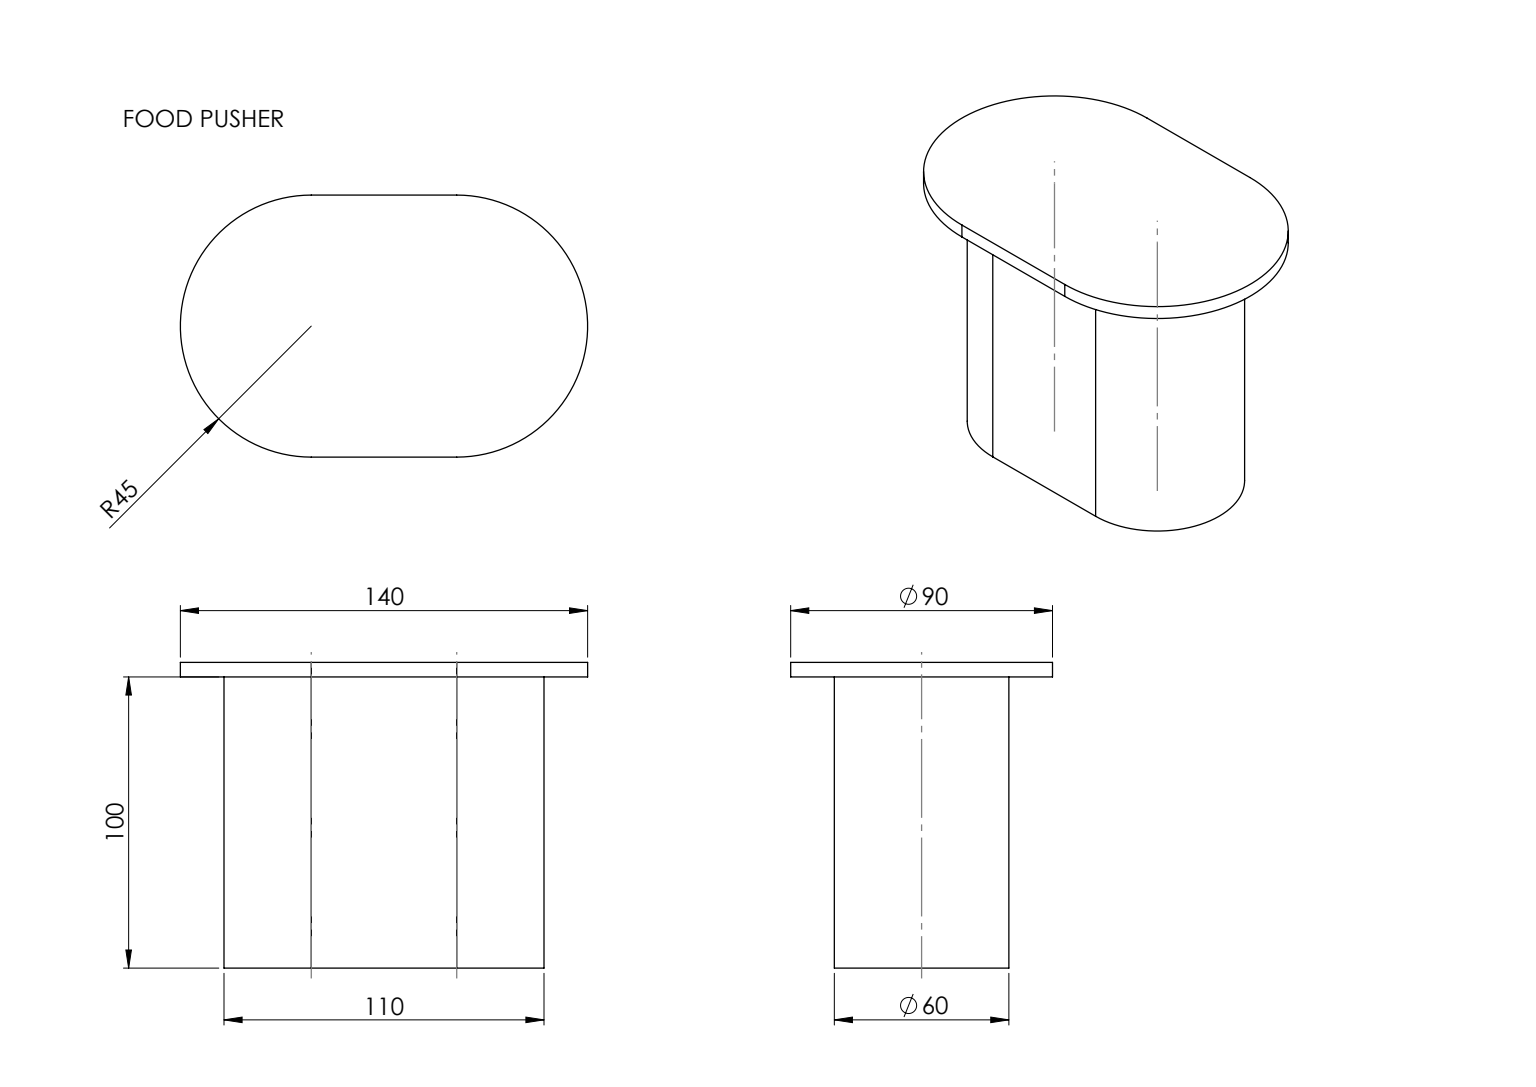
ISO-10303-21;
HEADER;
FILE_DESCRIPTION (('STEP AP214'),
    '1' );
FILE_NAME ('Food Pusher.step',
    '2026-10-08T14:59:03',
    ( '' ),
    ( '' ),
    'SwSTEP 2.0',
    'SolidWorks 2026',
    '' );
FILE_SCHEMA (( 'AUTOMOTIVE_DESIGN' ));
ENDSEC;

DATA;
#34=DIRECTION ( 'NONE',  ( 0.000000000000000000, -0.000000000000000000, 1.000000000000000000 ) ) ;
#70=CARTESIAN_POINT ( 'NONE',  ( -25.00000000000000000, 347.0000000000000568, -88.00000000000000000 ) ) ;
#77=PRESENTATION_STYLE_ASSIGNMENT (( #1089 ) ) ;
#97=CARTESIAN_POINT ( 'NONE',  ( 25.00000000000000000, 445.0000000000000568, -59.99999999999999289 ) ) ;
#102=PRODUCT ( 'Food Pusher', 'Food Pusher', '', ( #178 ) ) ;
#125=AXIS2_PLACEMENT_3D ( 'NONE', #9417, #9481, #11434 ) ;
#140=EDGE_CURVE ( 'NONE', #6671, #381, #10679, .T. ) ;
#178=PRODUCT_CONTEXT ( 'NONE', #12278, 'mechanical' ) ;
#190=DIRECTION ( 'NONE',  ( 0.000000000000000000, 1.000000000000000000, 0.000000000000000000 ) ) ;
#266=ORIENTED_EDGE ( 'NONE', *, *, #6038, .T. ) ;
#269=PRODUCT_DEFINITION_CONTEXT ( 'detailed design', #4862, 'design' ) ;
#304=EDGE_CURVE ( 'NONE', #3140, #9041, #7672, .T. ) ;
#351=EDGE_CURVE ( 'NONE', #5322, #7972, #10426, .T. ) ;
#367=LINE ( 'NONE', #11973, #3584 ) ;
#381=VERTEX_POINT ( 'NONE', #5888 ) ;
#385=AXIS2_PLACEMENT_3D ( 'NONE', #9164, #2752, #5571 ) ;
#431=ORIENTED_EDGE ( 'NONE', *, *, #7084, .F. ) ;
#458=CARTESIAN_POINT ( 'NONE',  ( -25.00000000000000000, 345.0000000000000568, -29.99999999999999289 ) ) ;
#475=CARTESIAN_POINT ( 'NONE',  ( 25.00000000000000355, 347.0000000000000568, -31.99999999999998579 ) ) ;
#481=ADVANCED_FACE ( 'NONE', ( #10318 ), #11460, .T. ) ;
#530=UNCERTAINTY_MEASURE_WITH_UNIT (LENGTH_MEASURE( 1.000000000000000082E-05 ), #1165, 'distance_accuracy_value', 'NONE');
#538=EDGE_CURVE ( 'NONE', #3006, #5730, #8937, .T. ) ;
#543=BREP_WITH_VOIDS ( 'NONE', #9857, ( #2440 ) );
#547=ORIENTED_EDGE ( 'NONE', *, *, #6712, .T. ) ;
#549=LINE ( 'NONE', #7222, #4086 ) ;
#581=ORIENTED_EDGE ( 'NONE', *, *, #4046, .F. ) ;
#591=ORIENTED_EDGE ( 'NONE', *, *, #140, .T. ) ;
#598=DIRECTION ( 'NONE',  ( 1.000000000000000000, 0.000000000000000000, 6.938893903907229610E-17 ) ) ;
#684=CARTESIAN_POINT ( 'NONE',  ( 25.00000000000000000, 445.0000000000000568, -59.99999999999999289 ) ) ;
#689=LINE ( 'NONE', #7424, #4842 ) ;
#727=AXIS2_PLACEMENT_3D ( 'NONE', #9151, #8407, #2620 ) ;
#755=FACE_OUTER_BOUND ( 'NONE', #1895, .T. ) ;
#758=CARTESIAN_POINT ( 'NONE',  ( -25.00000000000000000, 345.0000000000000568, -90.00000000000000000 ) ) ;
#776=MECHANICAL_DESIGN_GEOMETRIC_PRESENTATION_REPRESENTATION('',(#5155),#10705);
#836=ORIENTED_EDGE ( 'NONE', *, *, #7826, .F. ) ;
#837=DIRECTION ( 'NONE',  ( 0.000000000000000000, -0.000000000000000000, 1.000000000000000000 ) ) ;
#869=PRODUCT_DEFINITION ( 'UNKNOWN', '', #3750, #269 ) ;
#915=LINE ( 'NONE', #11450, #4998 ) ;
#940=LINE ( 'NONE', #12287, #7026 ) ;
#961=ORIENTED_EDGE ( 'NONE', *, *, #5528, .F. ) ;
#999=CARTESIAN_POINT ( 'NONE',  ( -25.00000000000000000, 445.0000000000000568, -29.99999999999999289 ) ) ;
#1065=CYLINDRICAL_SURFACE ( 'NONE', #6806, 44.99999999999999289 ) ;
#1077=FACE_OUTER_BOUND ( 'NONE', #5495, .T. ) ;
#1089=SURFACE_STYLE_USAGE ( .BOTH. , #2893 ) ;
#1095=VERTEX_POINT ( 'NONE', #1645 ) ;
#1102=AXIS2_PLACEMENT_3D ( 'NONE', #5202, #8863, #11996 ) ;
#1119=VECTOR ( 'NONE', #10886, 1000.000000000000000 ) ;
#1120=ORIENTED_EDGE ( 'NONE', *, *, #11826, .T. ) ;
#1165=( LENGTH_UNIT ( ) NAMED_UNIT ( * ) SI_UNIT ( .MILLI., .METRE. ) );
#1181=ADVANCED_FACE ( 'NONE', ( #10357 ), #10419, .F. ) ;
#1201=CARTESIAN_POINT ( 'NONE',  ( 25.00000000000000000, 570.2996408614167194, -59.99999999999999289 ) ) ;
#1219=DIRECTION ( 'NONE',  ( 0.000000000000000000, 0.000000000000000000, 1.000000000000000000 ) ) ;
#1241=ORIENTED_EDGE ( 'NONE', *, *, #2131, .F. ) ;
#1287=CARTESIAN_POINT ( 'NONE',  ( -25.00000000000000000, 570.2996408614167194, -29.99999999999999289 ) ) ;
#1303=ORIENTED_EDGE ( 'NONE', *, *, #5273, .F. ) ;
#1345=EDGE_CURVE ( 'NONE', #11537, #3527, #3608, .T. ) ;
#1374=VERTEX_POINT ( 'NONE', #8728 ) ;
#1396=EDGE_CURVE ( 'NONE', #11537, #1374, #6932, .T. ) ;
#1458=ORIENTED_EDGE ( 'NONE', *, *, #7606, .F. ) ;
#1492=DIRECTION ( 'NONE',  ( 1.000000000000000000, 0.000000000000000000, -0.000000000000000000 ) ) ;
#1503=EDGE_LOOP ( 'NONE', ( #8693, #4343, #10905, #836 ) ) ;
#1508=ORIENTED_EDGE ( 'NONE', *, *, #4461, .F. ) ;
#1585=( GEOMETRIC_REPRESENTATION_CONTEXT ( 3 ) GLOBAL_UNCERTAINTY_ASSIGNED_CONTEXT ( ( #530 ) ) GLOBAL_UNIT_ASSIGNED_CONTEXT ( ( #1165, #7827, #5035 ) ) REPRESENTATION_CONTEXT ( 'NONE', 'WORKASPACE' ) );
#1599=VECTOR ( 'NONE', #1889, 1000.000000000000000 ) ;
#1601=DIRECTION ( 'NONE',  ( 1.000000000000000000, -0.000000000000000000, 6.938893903907228378E-17 ) ) ;
#1612=AXIS2_PLACEMENT_3D ( 'NONE', #9562, #7823, #5032 ) ;
#1636=EDGE_LOOP ( 'NONE', ( #5230, #2543, #266, #6949 ) ) ;
#1645=CARTESIAN_POINT ( 'NONE',  ( 25.00000000000000355, 445.0000000000000568, -31.99999999999998579 ) ) ;
#1650=CARTESIAN_POINT ( 'NONE',  ( -25.00000000000000000, 450.0000000000000568, -14.99999999999999289 ) ) ;
#1651=VECTOR ( 'NONE', #598, 1000.000000000000000 ) ;
#1670=CARTESIAN_POINT ( 'NONE',  ( -25.00000000000000000, 445.0000000000000568, -59.99999999999999289 ) ) ;
#1734=VERTEX_POINT ( 'NONE', #758 ) ;
#1741=ADVANCED_FACE ( 'NONE', ( #7427 ), #8571, .F. ) ;
#1743=DIRECTION ( 'NONE',  ( 0.000000000000000000, 0.000000000000000000, 1.000000000000000000 ) ) ;
#1772=ORIENTED_EDGE ( 'NONE', *, *, #6771, .T. ) ;
#1777=ORIENTED_EDGE ( 'NONE', *, *, #8505, .T. ) ;
#1807=EDGE_LOOP ( 'NONE', ( #2058, #5789, #5095, #6562 ) ) ;
#1809=PLANE ( 'NONE',  #727 ) ;
#1819=VECTOR ( 'NONE', #2010, 1000.000000000000000 ) ;
#1848=DIRECTION ( 'NONE',  ( -0.000000000000000000, -1.000000000000000000, -0.000000000000000000 ) ) ;
#1875=CIRCLE ( 'NONE', #11248, 30.00000000000000355 ) ;
#1889=DIRECTION ( 'NONE',  ( -1.000000000000000000, 0.000000000000000000, 0.000000000000000000 ) ) ;
#1895=EDGE_LOOP ( 'NONE', ( #3084, #6423, #581, #4488 ) ) ;
#1908=ORIENTED_EDGE ( 'NONE', *, *, #1345, .T. ) ;
#1955=DIRECTION ( 'NONE',  ( -0.000000000000000000, -1.000000000000000000, -0.000000000000000000 ) ) ;
#2010=DIRECTION ( 'NONE',  ( -0.000000000000000000, -1.000000000000000000, -0.000000000000000000 ) ) ;
#2020=AXIS2_PLACEMENT_3D ( 'NONE', #97, #11523, #34 ) ;
#2058=ORIENTED_EDGE ( 'NONE', *, *, #5528, .T. ) ;
#2070=EDGE_LOOP ( 'NONE', ( #3023, #6435, #6345, #7354 ) ) ;
#2113=VERTEX_POINT ( 'NONE', #3709 ) ;
#2131=EDGE_CURVE ( 'NONE', #10138, #2113, #915, .T. ) ;
#2158=EDGE_CURVE ( 'NONE', #1095, #5322, #3373, .T. ) ;
#2170=EDGE_LOOP ( 'NONE', ( #1120, #3244, #10555, #5195 ) ) ;
#2190=CARTESIAN_POINT ( 'NONE',  ( 25.00000000000000000, 450.0000000000000568, -14.99999999999998934 ) ) ;
#2237=CARTESIAN_POINT ( 'NONE',  ( -24.99999999999999645, 450.0000000000000568, -105.0000000000000000 ) ) ;
#2338=FILL_AREA_STYLE_COLOUR ( '', #6280 ) ;
#2364=ADVANCED_FACE ( 'NONE', ( #9805 ), #3210, .T. ) ;
#2396=AXIS2_PLACEMENT_3D ( 'NONE', #8499, #10502, #12320 ) ;
#2440=ORIENTED_CLOSED_SHELL ( 'NONE', *, #12071, .F. );
#2466=ADVANCED_FACE ( 'NONE', ( #6560 ), #4626, .T. ) ;
#2543=ORIENTED_EDGE ( 'NONE', *, *, #9022, .T. ) ;
#2565=EDGE_LOOP ( 'NONE', ( #6905, #5701, #7059, #11308 ) ) ;
#2620=DIRECTION ( 'NONE',  ( 0.000000000000000000, -0.000000000000000000, 1.000000000000000000 ) ) ;
#2647=CARTESIAN_POINT ( 'NONE',  ( -25.00000000000000000, 347.0000000000000568, -59.99999999999999289 ) ) ;
#2657=ADVANCED_FACE ( 'NONE', ( #5934 ), #8665, .F. ) ;
#2699=ORIENTED_EDGE ( 'NONE', *, *, #2131, .T. ) ;
#2752=DIRECTION ( 'NONE',  ( 6.938893903907228378E-17, 0.000000000000000000, -1.000000000000000000 ) ) ;
#2767=DIRECTION ( 'NONE',  ( 0.000000000000000000, 0.000000000000000000, 1.000000000000000000 ) ) ;
#2783=DIRECTION ( 'NONE',  ( 0.000000000000000000, 0.000000000000000000, 1.000000000000000000 ) ) ;
#2795=VECTOR ( 'NONE', #3014, 1000.000000000000000 ) ;
#2811=ORIENTED_EDGE ( 'NONE', *, *, #4159, .F. ) ;
#2814=AXIS2_PLACEMENT_3D ( 'NONE', #4066, #190, #5937 ) ;
#2824=ORIENTED_EDGE ( 'NONE', *, *, #304, .F. ) ;
#2831=EDGE_LOOP ( 'NONE', ( #7123, #8086, #11427, #1508 ) ) ;
#2832=FILL_AREA_STYLE ('',( #5769 ) ) ;
#2835=AXIS2_PLACEMENT_3D ( 'NONE', #6137, #6950, #1219 ) ;
#2837=CARTESIAN_POINT ( 'NONE',  ( 25.00000000000000000, 445.0000000000000568, -59.99999999999999289 ) ) ;
#2893=SURFACE_SIDE_STYLE ('',( #6634 ) ) ;
#2902=DIRECTION ( 'NONE',  ( -0.000000000000000000, -1.000000000000000000, -0.000000000000000000 ) ) ;
#2931=LINE ( 'NONE', #3988, #5877 ) ;
#2943=CARTESIAN_POINT ( 'NONE',  ( -24.99999999999999289, 450.0000000000000568, -14.99999999999999289 ) ) ;
#2957=SHAPE_REPRESENTATION_RELATIONSHIP ( 'NONE' , 'NONE' ,  #8876, #6166 ) ;
#3006=VERTEX_POINT ( 'NONE', #999 ) ;
#3014=DIRECTION ( 'NONE',  ( -1.000000000000000000, 0.000000000000000000, 0.000000000000000000 ) ) ;
#3023=ORIENTED_EDGE ( 'NONE', *, *, #7075, .T. ) ;
#3084=ORIENTED_EDGE ( 'NONE', *, *, #2158, .T. ) ;
#3105=ORIENTED_EDGE ( 'NONE', *, *, #11826, .F. ) ;
#3127=ORIENTED_EDGE ( 'NONE', *, *, #1396, .F. ) ;
#3140=VERTEX_POINT ( 'NONE', #4795 ) ;
#3155=DIRECTION ( 'NONE',  ( -0.000000000000000000, -1.000000000000000000, -0.000000000000000000 ) ) ;
#3210=PLANE ( 'NONE',  #10957 ) ;
#3225=DIRECTION ( 'NONE',  ( 0.000000000000000000, -0.000000000000000000, 1.000000000000000000 ) ) ;
#3244=ORIENTED_EDGE ( 'NONE', *, *, #8505, .F. ) ;
#3249=DIRECTION ( 'NONE',  ( 0.000000000000000000, 0.000000000000000000, -1.000000000000000000 ) ) ;
#3251=CIRCLE ( 'NONE', #4048, 45.00000000000000000 ) ;
#3291=VECTOR ( 'NONE', #5624, 1000.000000000000000 ) ;
#3305=AXIS2_PLACEMENT_3D ( 'NONE', #9278, #11039, #5620 ) ;
#3318=DIRECTION ( 'NONE',  ( -0.000000000000000000, -1.000000000000000000, -0.000000000000000000 ) ) ;
#3326=DIRECTION ( 'NONE',  ( -0.000000000000000000, -1.000000000000000000, -0.000000000000000000 ) ) ;
#3357=EDGE_CURVE ( 'NONE', #5022, #9737, #12322, .T. ) ;
#3373=CIRCLE ( 'NONE', #2396, 28.00000000000000355 ) ;
#3436=VERTEX_POINT ( 'NONE', #5463 ) ;
#3456=CIRCLE ( 'NONE', #9811, 45.00000000000000000 ) ;
#3480=DIRECTION ( 'NONE',  ( 0.000000000000000000, 0.000000000000000000, 1.000000000000000000 ) ) ;
#3527=VERTEX_POINT ( 'NONE', #3959 ) ;
#3535=CARTESIAN_POINT ( 'NONE',  ( -25.00000000000000000, 347.0000000000000568, -31.99999999999999289 ) ) ;
#3554=CYLINDRICAL_SURFACE ( 'NONE', #5641, 28.00000000000000355 ) ;
#3558=CARTESIAN_POINT ( 'NONE',  ( 25.00000000000000000, 347.0000000000000568, -59.99999999999999289 ) ) ;
#3584=VECTOR ( 'NONE', #4173, 1000.000000000000000 ) ;
#3608=CIRCLE ( 'NONE', #2814, 45.00000000000000000 ) ;
#3620=FACE_OUTER_BOUND ( 'NONE', #7230, .T. ) ;
#3645=( LENGTH_UNIT ( ) NAMED_UNIT ( * ) SI_UNIT ( .MILLI., .METRE. ) );
#3649=CARTESIAN_POINT ( 'NONE',  ( -25.00000000000000000, 445.0000000000000568, -31.99999999999999289 ) ) ;
#3695=LINE ( 'NONE', #6513, #8088 ) ;
#3701=( NAMED_UNIT ( * ) SI_UNIT ( $, .STERADIAN. ) SOLID_ANGLE_UNIT ( ) );
#3709=CARTESIAN_POINT ( 'NONE',  ( -25.00000000000000000, 445.0000000000000568, -14.99999999999999289 ) ) ;
#3711=LINE ( 'NONE', #6336, #11290 ) ;
#3718=ADVANCED_FACE ( 'NONE', ( #1077 ), #4753, .T. ) ;
#3729=CARTESIAN_POINT ( 'NONE',  ( -25.00000000000000000, 445.0000000000000568, -29.99999999999999289 ) ) ;
#3735=VERTEX_POINT ( 'NONE', #4885 ) ;
#3750=PRODUCT_DEFINITION_FORMATION_WITH_SPECIFIED_SOURCE ( 'ANY', '', #102, .NOT_KNOWN. ) ;
#3777=UNCERTAINTY_MEASURE_WITH_UNIT (LENGTH_MEASURE( 1.000000000000000082E-05 ), #3645, 'distance_accuracy_value', 'NONE');
#3847=CARTESIAN_POINT ( 'NONE',  ( -25.00000000000000000, 445.0000000000000568, -59.99999999999999289 ) ) ;
#3888=CYLINDRICAL_SURFACE ( 'NONE', #125, 30.00000000000000711 ) ;
#3903=AXIS2_PLACEMENT_3D ( 'NONE', #1201, #7741, #11555 ) ;
#3910=AXIS2_PLACEMENT_3D ( 'NONE', #3558, #5558, #9397 ) ;
#3914=CARTESIAN_POINT ( 'NONE',  ( -25.00000000000000000, 445.0000000000000568, -59.99999999999999289 ) ) ;
#3959=CARTESIAN_POINT ( 'NONE',  ( 25.00000000000000355, 450.0000000000000568, -105.0000000000000000 ) ) ;
#3969=ADVANCED_FACE ( 'NONE', ( #3620 ), #1809, .T. ) ;
#3988=CARTESIAN_POINT ( 'NONE',  ( 25.00000000000000355, 450.0000000000000568, -105.0000000000000000 ) ) ;
#4022=ADVANCED_FACE ( 'NONE', ( #4427 ), #6548, .F. ) ;
#4046=EDGE_CURVE ( 'NONE', #5931, #8932, #9265, .T. ) ;
#4048=AXIS2_PLACEMENT_3D ( 'NONE', #7472, #9261, #3480 ) ;
#4066=CARTESIAN_POINT ( 'NONE',  ( 25.00000000000000000, 450.0000000000000568, -59.99999999999999289 ) ) ;
#4086=VECTOR ( 'NONE', #10264, 1000.000000000000000 ) ;
#4159=EDGE_CURVE ( 'NONE', #3527, #3436, #2931, .T. ) ;
#4173=DIRECTION ( 'NONE',  ( -0.000000000000000000, -1.000000000000000000, -0.000000000000000000 ) ) ;
#4186=CYLINDRICAL_SURFACE ( 'NONE', #6111, 28.00000000000000355 ) ;
#4214=SURFACE_STYLE_USAGE ( .BOTH. , #8995 ) ;
#4262=LINE ( 'NONE', #458, #10394 ) ;
#4268=AXIS2_PLACEMENT_3D ( 'NONE', #9352, #11369, #837 ) ;
#4343=ORIENTED_EDGE ( 'NONE', *, *, #6771, .F. ) ;
#4345=ORIENTED_EDGE ( 'NONE', *, *, #5273, .T. ) ;
#4427=FACE_OUTER_BOUND ( 'NONE', #2565, .T. ) ;
#4461=EDGE_CURVE ( 'NONE', #5322, #8932, #549, .T. ) ;
#4463=DIRECTION ( 'NONE',  ( 0.000000000000000000, 1.000000000000000000, 0.000000000000000000 ) ) ;
#4488=ORIENTED_EDGE ( 'NONE', *, *, #7328, .F. ) ;
#4546=CARTESIAN_POINT ( 'NONE',  ( 25.00000000000000000, 570.2996408614167194, -59.99999999999999289 ) ) ;
#4554=LINE ( 'NONE', #8468, #3291 ) ;
#4626=PLANE ( 'NONE',  #385 ) ;
#4753=CYLINDRICAL_SURFACE ( 'NONE', #3903, 30.00000000000000711 ) ;
#4795=CARTESIAN_POINT ( 'NONE',  ( 25.00000000000000355, 445.0000000000000568, -90.00000000000000000 ) ) ;
#4842=VECTOR ( 'NONE', #8282, 1000.000000000000000 ) ;
#4862=APPLICATION_CONTEXT ( 'automotive_design' ) ;
#4869=DIRECTION ( 'NONE',  ( -0.000000000000000000, -1.000000000000000000, -0.000000000000000000 ) ) ;
#4885=CARTESIAN_POINT ( 'NONE',  ( -24.99999999999999645, 445.0000000000000568, -105.0000000000000000 ) ) ;
#4893=( NAMED_UNIT ( * ) PLANE_ANGLE_UNIT ( ) SI_UNIT ( $, .RADIAN. ) );
#4930=ORIENTED_EDGE ( 'NONE', *, *, #7084, .T. ) ;
#4931=SHAPE_DEFINITION_REPRESENTATION ( #5691, #8876 ) ;
#4994=ORIENTED_EDGE ( 'NONE', *, *, #2158, .F. ) ;
#4998=VECTOR ( 'NONE', #2902, 1000.000000000000000 ) ;
#5022=VERTEX_POINT ( 'NONE', #70 ) ;
#5032=DIRECTION ( 'NONE',  ( 1.000000000000000000, 0.000000000000000000, 0.000000000000000000 ) ) ;
#5035=( NAMED_UNIT ( * ) SI_UNIT ( $, .STERADIAN. ) SOLID_ANGLE_UNIT ( ) );
#5038=DIRECTION ( 'NONE',  ( -0.000000000000000000, -1.000000000000000000, -0.000000000000000000 ) ) ;
#5095=ORIENTED_EDGE ( 'NONE', *, *, #7266, .T. ) ;
#5155=STYLED_ITEM ( 'NONE', ( #77 ), #6166 ) ;
#5195=ORIENTED_EDGE ( 'NONE', *, *, #1396, .T. ) ;
#5202=CARTESIAN_POINT ( 'NONE',  ( 25.00000000000000000, 570.2996408614167194, -88.00000000000000000 ) ) ;
#5204=EDGE_LOOP ( 'NONE', ( #1908, #6125, #4930, #10213 ) ) ;
#5213=AXIS2_PLACEMENT_3D ( 'NONE', #10780, #6167, #1492 ) ;
#5230=ORIENTED_EDGE ( 'NONE', *, *, #7266, .F. ) ;
#5273=EDGE_CURVE ( 'NONE', #2113, #1374, #4554, .T. ) ;
#5295=ORIENTED_EDGE ( 'NONE', *, *, #4046, .T. ) ;
#5322=VERTEX_POINT ( 'NONE', #6860 ) ;
#5389=CARTESIAN_POINT ( 'NONE',  ( -25.00000000000000000, 445.0000000000000568, -88.00000000000000000 ) ) ;
#5404=LINE ( 'NONE', #9118, #1651 ) ;
#5463=CARTESIAN_POINT ( 'NONE',  ( -24.99999999999999645, 450.0000000000000568, -105.0000000000000000 ) ) ;
#5480=DIRECTION ( 'NONE',  ( 0.000000000000000000, 1.000000000000000000, 0.000000000000000000 ) ) ;
#5483=CARTESIAN_POINT ( 'NONE',  ( 25.00000000000000355, 345.0000000000000568, -90.00000000000000000 ) ) ;
#5495=EDGE_LOOP ( 'NONE', ( #961, #591, #8838, #5936 ) ) ;
#5528=EDGE_CURVE ( 'NONE', #6671, #3140, #9021, .T. ) ;
#5550=ORIENTED_EDGE ( 'NONE', *, *, #8649, .F. ) ;
#5558=DIRECTION ( 'NONE',  ( 0.000000000000000000, 1.000000000000000000, 0.000000000000000000 ) ) ;
#5571=DIRECTION ( 'NONE',  ( -1.000000000000000000, 0.000000000000000000, -6.938893903907228378E-17 ) ) ;
#5598=EDGE_CURVE ( 'NONE', #3436, #3735, #8087, .T. ) ;
#5601=DIRECTION ( 'NONE',  ( 0.000000000000000000, 0.000000000000000000, -1.000000000000000000 ) ) ;
#5620=DIRECTION ( 'NONE',  ( -1.000000000000000000, 0.000000000000000000, -6.938893903907228378E-17 ) ) ;
#5624=DIRECTION ( 'NONE',  ( 1.000000000000000000, 0.000000000000000000, 6.938893903907229610E-17 ) ) ;
#5641=AXIS2_PLACEMENT_3D ( 'NONE', #4546, #7600, #6361 ) ;
#5691=PRODUCT_DEFINITION_SHAPE ( 'NONE', 'NONE',  #869 ) ;
#5701=ORIENTED_EDGE ( 'NONE', *, *, #538, .T. ) ;
#5709=ORIENTED_EDGE ( 'NONE', *, *, #7328, .T. ) ;
#5730=VERTEX_POINT ( 'NONE', #9266 ) ;
#5735=VERTEX_POINT ( 'NONE', #5483 ) ;
#5769=FILL_AREA_STYLE_COLOUR ( '', #8936 ) ;
#5782=AXIS2_PLACEMENT_3D ( 'NONE', #684, #10272, #1743 ) ;
#5789=ORIENTED_EDGE ( 'NONE', *, *, #304, .T. ) ;
#5800=EDGE_LOOP ( 'NONE', ( #6656, #5709, #5550, #11223 ) ) ;
#5816=ORIENTED_EDGE ( 'NONE', *, *, #11731, .T. ) ;
#5849=AXIS2_PLACEMENT_3D ( 'NONE', #3914, #5907, #8755 ) ;
#5873=DIRECTION ( 'NONE',  ( -1.000000000000000000, 0.000000000000000000, 0.000000000000000000 ) ) ;
#5877=VECTOR ( 'NONE', #6730, 1000.000000000000000 ) ;
#5888=CARTESIAN_POINT ( 'NONE',  ( 25.00000000000000000, 345.0000000000000568, -29.99999999999998934 ) ) ;
#5907=DIRECTION ( 'NONE',  ( 0.000000000000000000, 1.000000000000000000, 0.000000000000000000 ) ) ;
#5931=VERTEX_POINT ( 'NONE', #475 ) ;
#5934=FACE_OUTER_BOUND ( 'NONE', #7350, .T. ) ;
#5936=ORIENTED_EDGE ( 'NONE', *, *, #11731, .F. ) ;
#5937=DIRECTION ( 'NONE',  ( 0.000000000000000000, 0.000000000000000000, 1.000000000000000000 ) ) ;
#5970=ADVANCED_FACE ( 'NONE', ( #10764 ), #7149, .F. ) ;
#6038=EDGE_CURVE ( 'NONE', #1734, #5730, #1875, .T. ) ;
#6062=VECTOR ( 'NONE', #11910, 1000.000000000000000 ) ;
#6087=VECTOR ( 'NONE', #3155, 1000.000000000000000 ) ;
#6104=ADVANCED_FACE ( 'NONE', ( #11875 ), #11749, .T. ) ;
#6111=AXIS2_PLACEMENT_3D ( 'NONE', #6123, #3318, #3249 ) ;
#6123=CARTESIAN_POINT ( 'NONE',  ( -25.00000000000000000, 570.2996408614167194, -59.99999999999999289 ) ) ;
#6125=ORIENTED_EDGE ( 'NONE', *, *, #4159, .T. ) ;
#6137=CARTESIAN_POINT ( 'NONE',  ( 25.00000000000000000, 345.0000000000000568, -59.99999999999999289 ) ) ;
#6154=EDGE_LOOP ( 'NONE', ( #10020, #1241, #431, #9354 ) ) ;
#6166=ADVANCED_BREP_SHAPE_REPRESENTATION ( '', ( #543, #1612 ), #9911 ) ;
#6167=DIRECTION ( 'NONE',  ( 0.000000000000000000, -0.000000000000000000, 1.000000000000000000 ) ) ;
#6199=DIRECTION ( 'NONE',  ( 0.000000000000000000, -0.000000000000000000, 1.000000000000000000 ) ) ;
#6200=DIRECTION ( 'NONE',  ( 0.000000000000000000, -0.000000000000000000, 1.000000000000000000 ) ) ;
#6280=COLOUR_RGB ( '', 0.31764706, 0.68627451, 0.89019608) ;
#6298=EDGE_CURVE ( 'NONE', #7972, #5022, #6380, .T. ) ;
#6336=CARTESIAN_POINT ( 'NONE',  ( -25.00000000000000000, 347.0000000000000568, -31.99999999999999289 ) ) ;
#6345=ORIENTED_EDGE ( 'NONE', *, *, #3357, .F. ) ;
#6361=DIRECTION ( 'NONE',  ( 0.000000000000000000, 0.000000000000000000, -1.000000000000000000 ) ) ;
#6362=EDGE_LOOP ( 'NONE', ( #6970, #11839, #2811, #1777 ) ) ;
#6380=LINE ( 'NONE', #11876, #11261 ) ;
#6423=ORIENTED_EDGE ( 'NONE', *, *, #4461, .T. ) ;
#6424=AXIS2_PLACEMENT_3D ( 'NONE', #2837, #10438, #6199 ) ;
#6426=CARTESIAN_POINT ( 'NONE',  ( 25.00000000000000000, 445.0000000000000568, -29.99999999999998934 ) ) ;
#6435=ORIENTED_EDGE ( 'NONE', *, *, #8750, .T. ) ;
#6447=DIRECTION ( 'NONE',  ( 1.000000000000000000, -0.000000000000000000, 6.938893903907228378E-17 ) ) ;
#6508=VERTEX_POINT ( 'NONE', #8095 ) ;
#6513=CARTESIAN_POINT ( 'NONE',  ( -25.00000000000000000, 445.0000000000000568, -31.99999999999999289 ) ) ;
#6548=PLANE ( 'NONE',  #3305 ) ;
#6560=FACE_OUTER_BOUND ( 'NONE', #5800, .T. ) ;
#6562=ORIENTED_EDGE ( 'NONE', *, *, #11915, .T. ) ;
#6572=( NAMED_UNIT ( * ) PLANE_ANGLE_UNIT ( ) SI_UNIT ( $, .RADIAN. ) );
#6634=SURFACE_STYLE_FILL_AREA ( #2832 ) ;
#6649=CARTESIAN_POINT ( 'NONE',  ( -25.00000000000000000, 450.0000000000000568, -59.99999999999999289 ) ) ;
#6656=ORIENTED_EDGE ( 'NONE', *, *, #8954, .T. ) ;
#6671=VERTEX_POINT ( 'NONE', #6426 ) ;
#6712=EDGE_CURVE ( 'NONE', #8932, #5022, #940, .T. ) ;
#6730=DIRECTION ( 'NONE',  ( -1.000000000000000000, 0.000000000000000000, 0.000000000000000000 ) ) ;
#6736=CARTESIAN_POINT ( 'NONE',  ( 25.00000000000000000, 450.0000000000000568, -59.99999999999999289 ) ) ;
#6743=DIRECTION ( 'NONE',  ( 6.938893903907229610E-17, 0.000000000000000000, -1.000000000000000000 ) ) ;
#6756=( LENGTH_UNIT ( ) NAMED_UNIT ( * ) SI_UNIT ( .MILLI., .METRE. ) );
#6770=ADVANCED_FACE ( 'NONE', ( #755 ), #3554, .F. ) ;
#6771=EDGE_CURVE ( 'NONE', #5735, #1734, #689, .T. ) ;
#6779=VECTOR ( 'NONE', #11345, 1000.000000000000000 ) ;
#6806=AXIS2_PLACEMENT_3D ( 'NONE', #6736, #4869, #11418 ) ;
#6858=ORIENTED_EDGE ( 'NONE', *, *, #3357, .T. ) ;
#6860=CARTESIAN_POINT ( 'NONE',  ( 25.00000000000000355, 445.0000000000000568, -88.00000000000000000 ) ) ;
#6875=EDGE_LOOP ( 'NONE', ( #2824, #5816, #1772, #10024 ) ) ;
#6902=SURFACE_STYLE_FILL_AREA ( #8813 ) ;
#6905=ORIENTED_EDGE ( 'NONE', *, *, #11915, .F. ) ;
#6932=LINE ( 'NONE', #2190, #1819 ) ;
#6938=CARTESIAN_POINT ( 'NONE',  ( 25.00000000000000355, 445.0000000000000568, -105.0000000000000000 ) ) ;
#6941=CARTESIAN_POINT ( 'NONE',  ( 25.00000000000000000, 570.2996408614167194, -29.99999999999998934 ) ) ;
#6949=ORIENTED_EDGE ( 'NONE', *, *, #538, .F. ) ;
#6950=DIRECTION ( 'NONE',  ( 0.000000000000000000, 1.000000000000000000, 0.000000000000000000 ) ) ;
#6969=VECTOR ( 'NONE', #5873, 1000.000000000000000 ) ;
#6970=ORIENTED_EDGE ( 'NONE', *, *, #10307, .T. ) ;
#6978=PLANE ( 'NONE',  #5213 ) ;
#7024=DIRECTION ( 'NONE',  ( 1.000000000000000000, 0.000000000000000000, -0.000000000000000000 ) ) ;
#7026=VECTOR ( 'NONE', #7483, 1000.000000000000000 ) ;
#7059=ORIENTED_EDGE ( 'NONE', *, *, #7826, .T. ) ;
#7075=EDGE_CURVE ( 'NONE', #7972, #7578, #9405, .T. ) ;
#7084=EDGE_CURVE ( 'NONE', #3436, #10138, #3251, .T. ) ;
#7123=ORIENTED_EDGE ( 'NONE', *, *, #351, .T. ) ;
#7149=PLANE ( 'NONE',  #10234 ) ;
#7155=EDGE_LOOP ( 'NONE', ( #3105, #1303, #7287, #8340 ) ) ;
#7222=CARTESIAN_POINT ( 'NONE',  ( 25.00000000000000355, 570.2996408614167194, -88.00000000000000000 ) ) ;
#7230=EDGE_LOOP ( 'NONE', ( #6858, #9675, #5295, #547 ) ) ;
#7232=CIRCLE ( 'NONE', #5849, 30.00000000000000355 ) ;
#7266=EDGE_CURVE ( 'NONE', #9041, #3006, #7232, .T. ) ;
#7287=ORIENTED_EDGE ( 'NONE', *, *, #7299, .F. ) ;
#7299=EDGE_CURVE ( 'NONE', #3735, #2113, #3456, .T. ) ;
#7328=EDGE_CURVE ( 'NONE', #1095, #5931, #10003, .T. ) ;
#7350=EDGE_LOOP ( 'NONE', ( #4345, #3127, #1458, #2699 ) ) ;
#7354=ORIENTED_EDGE ( 'NONE', *, *, #6298, .F. ) ;
#7424=CARTESIAN_POINT ( 'NONE',  ( 25.00000000000000000, 345.0000000000000568, -90.00000000000000000 ) ) ;
#7427=FACE_OUTER_BOUND ( 'NONE', #8280, .T. ) ;
#7453=AXIS2_PLACEMENT_3D ( 'NONE', #11025, #9896, #10021 ) ;
#7472=CARTESIAN_POINT ( 'NONE',  ( -25.00000000000000000, 450.0000000000000568, -59.99999999999999289 ) ) ;
#7483=DIRECTION ( 'NONE',  ( -1.000000000000000000, 0.000000000000000000, 0.000000000000000000 ) ) ;
#7578=VERTEX_POINT ( 'NONE', #3649 ) ;
#7600=DIRECTION ( 'NONE',  ( -0.000000000000000000, -1.000000000000000000, -0.000000000000000000 ) ) ;
#7606=EDGE_CURVE ( 'NONE', #10138, #11537, #5404, .T. ) ;
#7672=LINE ( 'NONE', #10413, #6969 ) ;
#7741=DIRECTION ( 'NONE',  ( -0.000000000000000000, -1.000000000000000000, -0.000000000000000000 ) ) ;
#7762=ADVANCED_FACE ( 'NONE', ( #8745, #7820 ), #12319, .F. ) ;
#7820=FACE_OUTER_BOUND ( 'NONE', #7155, .T. ) ;
#7823=DIRECTION ( 'NONE',  ( 0.000000000000000000, 0.000000000000000000, 1.000000000000000000 ) ) ;
#7826=EDGE_CURVE ( 'NONE', #5730, #381, #4262, .T. ) ;
#7827=( NAMED_UNIT ( * ) PLANE_ANGLE_UNIT ( ) SI_UNIT ( $, .RADIAN. ) );
#7863=FACE_OUTER_BOUND ( 'NONE', #2070, .T. ) ;
#7865=STYLED_ITEM ( 'NONE', ( #8880 ), #543 ) ;
#7891=EDGE_CURVE ( 'NONE', #381, #5735, #11606, .T. ) ;
#7947=CARTESIAN_POINT ( 'NONE',  ( 25.00000000000000000, 570.2996408614167194, -90.00000000000000000 ) ) ;
#7972=VERTEX_POINT ( 'NONE', #5389 ) ;
#8007=CARTESIAN_POINT ( 'NONE',  ( 25.00000000000000355, 450.0000000000000568, -105.0000000000000000 ) ) ;
#8086=ORIENTED_EDGE ( 'NONE', *, *, #6298, .T. ) ;
#8087=LINE ( 'NONE', #2237, #6062 ) ;
#8088=VECTOR ( 'NONE', #6447, 1000.000000000000000 ) ;
#8095=CARTESIAN_POINT ( 'NONE',  ( 25.00000000000000355, 445.0000000000000568, -105.0000000000000000 ) ) ;
#8166=CARTESIAN_POINT ( 'NONE',  ( 25.00000000000000000, 450.0000000000000568, -14.99999999999998934 ) ) ;
#8245=LINE ( 'NONE', #12190, #10481 ) ;
#8278=LINE ( 'NONE', #3729, #6779 ) ;
#8280=EDGE_LOOP ( 'NONE', ( #11510, #4994, #8903, #10671 ) ) ;
#8282=DIRECTION ( 'NONE',  ( -1.000000000000000000, 0.000000000000000000, 0.000000000000000000 ) ) ;
#8313=DIRECTION ( 'NONE',  ( 0.000000000000000000, 1.000000000000000000, 0.000000000000000000 ) ) ;
#8340=ORIENTED_EDGE ( 'NONE', *, *, #10307, .F. ) ;
#8407=DIRECTION ( 'NONE',  ( 0.000000000000000000, 1.000000000000000000, 0.000000000000000000 ) ) ;
#8423=VECTOR ( 'NONE', #5038, 1000.000000000000000 ) ;
#8468=CARTESIAN_POINT ( 'NONE',  ( -24.99999999999999289, 445.0000000000000568, -14.99999999999999289 ) ) ;
#8499=CARTESIAN_POINT ( 'NONE',  ( 25.00000000000000000, 445.0000000000000568, -59.99999999999999289 ) ) ;
#8504=UNCERTAINTY_MEASURE_WITH_UNIT (LENGTH_MEASURE( 1.000000000000000082E-05 ), #6756, 'distance_accuracy_value', 'NONE');
#8505=EDGE_CURVE ( 'NONE', #3527, #6508, #9000, .T. ) ;
#8511=DIRECTION ( 'NONE',  ( 0.000000000000000000, 0.000000000000000000, 1.000000000000000000 ) ) ;
#8571=PLANE ( 'NONE',  #2020 ) ;
#8649=EDGE_CURVE ( 'NONE', #9737, #5931, #3711, .T. ) ;
#8665=PLANE ( 'NONE',  #10738 ) ;
#8693=ORIENTED_EDGE ( 'NONE', *, *, #6038, .F. ) ;
#8728=CARTESIAN_POINT ( 'NONE',  ( 25.00000000000000000, 445.0000000000000568, -14.99999999999998934 ) ) ;
#8745=FACE_BOUND ( 'NONE', #1807, .T. ) ;
#8750=EDGE_CURVE ( 'NONE', #7578, #9737, #11638, .T. ) ;
#8755=DIRECTION ( 'NONE',  ( 0.000000000000000000, 0.000000000000000000, 1.000000000000000000 ) ) ;
#8768=VECTOR ( 'NONE', #1955, 1000.000000000000000 ) ;
#8813=FILL_AREA_STYLE ('',( #2338 ) ) ;
#8838=ORIENTED_EDGE ( 'NONE', *, *, #7891, .T. ) ;
#8863=DIRECTION ( 'NONE',  ( 0.000000000000000000, -0.000000000000000000, 1.000000000000000000 ) ) ;
#8876=SHAPE_REPRESENTATION ( 'Food Pusher', ( #1612 ), #9911 ) ;
#8880=PRESENTATION_STYLE_ASSIGNMENT (( #4214 ) ) ;
#8903=ORIENTED_EDGE ( 'NONE', *, *, #8954, .F. ) ;
#8917=FACE_OUTER_BOUND ( 'NONE', #2170, .T. ) ;
#8932=VERTEX_POINT ( 'NONE', #11062 ) ;
#8936=COLOUR_RGB ( '', 0.31764706, 0.68627451, 0.89019608) ;
#8937=LINE ( 'NONE', #1287, #6087 ) ;
#8954=EDGE_CURVE ( 'NONE', #7578, #1095, #3695, .T. ) ;
#8995=SURFACE_SIDE_STYLE ('',( #6902 ) ) ;
#9000=LINE ( 'NONE', #8007, #1119 ) ;
#9016=FACE_OUTER_BOUND ( 'NONE', #6362, .T. ) ;
#9021=CIRCLE ( 'NONE', #7453, 30.00000000000000711 ) ;
#9022=EDGE_CURVE ( 'NONE', #9041, #1734, #8245, .T. ) ;
#9041=VERTEX_POINT ( 'NONE', #9357 ) ;
#9099=ADVANCED_FACE ( 'NONE', ( #9667 ), #3888, .T. ) ;
#9118=CARTESIAN_POINT ( 'NONE',  ( -24.99999999999999289, 450.0000000000000568, -14.99999999999999289 ) ) ;
#9151=CARTESIAN_POINT ( 'NONE',  ( -25.00000000000000000, 347.0000000000000568, -59.99999999999999289 ) ) ;
#9164=CARTESIAN_POINT ( 'NONE',  ( -25.00000000000000000, 570.2996408614167194, -31.99999999999999289 ) ) ;
#9261=DIRECTION ( 'NONE',  ( 0.000000000000000000, 1.000000000000000000, 0.000000000000000000 ) ) ;
#9265=CIRCLE ( 'NONE', #3910, 28.00000000000000355 ) ;
#9266=CARTESIAN_POINT ( 'NONE',  ( -25.00000000000000000, 345.0000000000000568, -29.99999999999999289 ) ) ;
#9278=CARTESIAN_POINT ( 'NONE',  ( -25.00000000000000000, 570.2996408614167194, -29.99999999999999289 ) ) ;
#9280=ADVANCED_FACE ( 'NONE', ( #7863 ), #4186, .F. ) ;
#9352=CARTESIAN_POINT ( 'NONE',  ( -25.00000000000000000, 345.0000000000000568, -59.99999999999999289 ) ) ;
#9354=ORIENTED_EDGE ( 'NONE', *, *, #5598, .T. ) ;
#9357=CARTESIAN_POINT ( 'NONE',  ( -25.00000000000000000, 445.0000000000000568, -90.00000000000000000 ) ) ;
#9397=DIRECTION ( 'NONE',  ( 0.000000000000000000, 0.000000000000000000, 1.000000000000000000 ) ) ;
#9405=CIRCLE ( 'NONE', #9612, 28.00000000000000355 ) ;
#9417=CARTESIAN_POINT ( 'NONE',  ( -25.00000000000000000, 570.2996408614167194, -59.99999999999999289 ) ) ;
#9481=DIRECTION ( 'NONE',  ( -0.000000000000000000, -1.000000000000000000, -0.000000000000000000 ) ) ;
#9529=ADVANCED_FACE ( 'NONE', ( #8917 ), #1065, .T. ) ;
#9562=CARTESIAN_POINT ( 'NONE',  ( 0.000000000000000000, 0.000000000000000000, 0.000000000000000000 ) ) ;
#9599=DIRECTION ( 'NONE',  ( -1.000000000000000000, 0.000000000000000000, -6.938893903907229610E-17 ) ) ;
#9612=AXIS2_PLACEMENT_3D ( 'NONE', #1670, #5480, #2783 ) ;
#9667=FACE_OUTER_BOUND ( 'NONE', #1636, .T. ) ;
#9675=ORIENTED_EDGE ( 'NONE', *, *, #8649, .T. ) ;
#9737=VERTEX_POINT ( 'NONE', #3535 ) ;
#9738=DIRECTION ( 'NONE',  ( 1.000000000000000000, 0.000000000000000000, 6.938893903907228378E-17 ) ) ;
#9805=FACE_OUTER_BOUND ( 'NONE', #5204, .T. ) ;
#9811=AXIS2_PLACEMENT_3D ( 'NONE', #3847, #10695, #8511 ) ;
#9857=CLOSED_SHELL ( 'NONE', ( #9529, #10919, #481, #2657, #2364, #7762, #1181, #3718, #4022, #9099, #5970 ) ) ;
#9878=CARTESIAN_POINT ( 'NONE',  ( 25.00000000000000355, 570.2996408614167194, -31.99999999999998579 ) ) ;
#9896=DIRECTION ( 'NONE',  ( 0.000000000000000000, 1.000000000000000000, 0.000000000000000000 ) ) ;
#9911=( GEOMETRIC_REPRESENTATION_CONTEXT ( 3 ) GLOBAL_UNCERTAINTY_ASSIGNED_CONTEXT ( ( #3777 ) ) GLOBAL_UNIT_ASSIGNED_CONTEXT ( ( #3645, #6572, #3701 ) ) REPRESENTATION_CONTEXT ( 'NONE', 'WORKASPACE' ) );
#10003=LINE ( 'NONE', #9878, #8423 ) ;
#10020=ORIENTED_EDGE ( 'NONE', *, *, #7299, .T. ) ;
#10021=DIRECTION ( 'NONE',  ( 0.000000000000000000, 0.000000000000000000, 1.000000000000000000 ) ) ;
#10024=ORIENTED_EDGE ( 'NONE', *, *, #9022, .F. ) ;
#10138=VERTEX_POINT ( 'NONE', #1650 ) ;
#10190=CARTESIAN_POINT ( 'NONE',  ( -25.00000000000000000, 345.0000000000000568, -59.99999999999999289 ) ) ;
#10213=ORIENTED_EDGE ( 'NONE', *, *, #7606, .T. ) ;
#10234=AXIS2_PLACEMENT_3D ( 'NONE', #7947, #3225, #7024 ) ;
#10264=DIRECTION ( 'NONE',  ( -0.000000000000000000, -1.000000000000000000, -0.000000000000000000 ) ) ;
#10272=DIRECTION ( 'NONE',  ( 0.000000000000000000, 1.000000000000000000, 0.000000000000000000 ) ) ;
#10307=EDGE_CURVE ( 'NONE', #6508, #3735, #11559, .T. ) ;
#10318=FACE_OUTER_BOUND ( 'NONE', #6154, .T. ) ;
#10357=FACE_OUTER_BOUND ( 'NONE', #1503, .T. ) ;
#10394=VECTOR ( 'NONE', #9738, 1000.000000000000000 ) ;
#10413=CARTESIAN_POINT ( 'NONE',  ( 25.00000000000000000, 445.0000000000000568, -90.00000000000000000 ) ) ;
#10419=PLANE ( 'NONE',  #4268 ) ;
#10426=LINE ( 'NONE', #10491, #1599 ) ;
#10431=( NAMED_UNIT ( * ) SI_UNIT ( $, .STERADIAN. ) SOLID_ANGLE_UNIT ( ) );
#10438=DIRECTION ( 'NONE',  ( 0.000000000000000000, 1.000000000000000000, 0.000000000000000000 ) ) ;
#10481=VECTOR ( 'NONE', #12004, 1000.000000000000000 ) ;
#10491=CARTESIAN_POINT ( 'NONE',  ( 25.00000000000000000, 445.0000000000000568, -88.00000000000000000 ) ) ;
#10502=DIRECTION ( 'NONE',  ( 0.000000000000000000, 1.000000000000000000, 0.000000000000000000 ) ) ;
#10555=ORIENTED_EDGE ( 'NONE', *, *, #1345, .F. ) ;
#10671=ORIENTED_EDGE ( 'NONE', *, *, #7075, .F. ) ;
#10679=LINE ( 'NONE', #6941, #8768 ) ;
#10695=DIRECTION ( 'NONE',  ( 0.000000000000000000, 1.000000000000000000, 0.000000000000000000 ) ) ;
#10705=( GEOMETRIC_REPRESENTATION_CONTEXT ( 3 ) GLOBAL_UNCERTAINTY_ASSIGNED_CONTEXT ( ( #8504 ) ) GLOBAL_UNIT_ASSIGNED_CONTEXT ( ( #6756, #4893, #10431 ) ) REPRESENTATION_CONTEXT ( 'NONE', 'WORKASPACE' ) );
#10733=MECHANICAL_DESIGN_GEOMETRIC_PRESENTATION_REPRESENTATION('',(#7865),#1585);
#10738=AXIS2_PLACEMENT_3D ( 'NONE', #2943, #6743, #9599 ) ;
#10764=FACE_OUTER_BOUND ( 'NONE', #6875, .T. ) ;
#10780=CARTESIAN_POINT ( 'NONE',  ( 25.00000000000000355, 450.0000000000000568, -105.0000000000000000 ) ) ;
#10808=CARTESIAN_POINT ( 'NONE',  ( 25.00000000000000000, 450.0000000000000568, -59.99999999999999289 ) ) ;
#10886=DIRECTION ( 'NONE',  ( -0.000000000000000000, -1.000000000000000000, -0.000000000000000000 ) ) ;
#10905=ORIENTED_EDGE ( 'NONE', *, *, #7891, .F. ) ;
#10919=ADVANCED_FACE ( 'NONE', ( #9016 ), #6978, .F. ) ;
#10957=AXIS2_PLACEMENT_3D ( 'NONE', #10808, #11882, #6200 ) ;
#11011=DIRECTION ( 'NONE',  ( 0.000000000000000000, 0.000000000000000000, 1.000000000000000000 ) ) ;
#11025=CARTESIAN_POINT ( 'NONE',  ( 25.00000000000000000, 445.0000000000000568, -59.99999999999999289 ) ) ;
#11039=DIRECTION ( 'NONE',  ( 6.938893903907228378E-17, 0.000000000000000000, -1.000000000000000000 ) ) ;
#11062=CARTESIAN_POINT ( 'NONE',  ( 25.00000000000000355, 347.0000000000000568, -88.00000000000000000 ) ) ;
#11223=ORIENTED_EDGE ( 'NONE', *, *, #8750, .F. ) ;
#11248=AXIS2_PLACEMENT_3D ( 'NONE', #10190, #4463, #11011 ) ;
#11261=VECTOR ( 'NONE', #3326, 1000.000000000000000 ) ;
#11290=VECTOR ( 'NONE', #1601, 1000.000000000000000 ) ;
#11308=ORIENTED_EDGE ( 'NONE', *, *, #140, .F. ) ;
#11345=DIRECTION ( 'NONE',  ( 1.000000000000000000, -0.000000000000000000, 6.938893903907228378E-17 ) ) ;
#11369=DIRECTION ( 'NONE',  ( 0.000000000000000000, 1.000000000000000000, 0.000000000000000000 ) ) ;
#11418=DIRECTION ( 'NONE',  ( 0.000000000000000000, 0.000000000000000000, -1.000000000000000000 ) ) ;
#11427=ORIENTED_EDGE ( 'NONE', *, *, #6712, .F. ) ;
#11434=DIRECTION ( 'NONE',  ( 0.000000000000000000, 0.000000000000000000, -1.000000000000000000 ) ) ;
#11450=CARTESIAN_POINT ( 'NONE',  ( -25.00000000000000000, 450.0000000000000568, -14.99999999999999289 ) ) ;
#11451=DIRECTION ( 'NONE',  ( -0.000000000000000000, -1.000000000000000000, -0.000000000000000000 ) ) ;
#11460=CYLINDRICAL_SURFACE ( 'NONE', #12064, 44.99999999999999289 ) ;
#11510=ORIENTED_EDGE ( 'NONE', *, *, #351, .F. ) ;
#11513=CARTESIAN_POINT ( 'NONE',  ( -25.00000000000000000, 570.2996408614167194, -31.99999999999999289 ) ) ;
#11523=DIRECTION ( 'NONE',  ( 0.000000000000000000, 1.000000000000000000, 0.000000000000000000 ) ) ;
#11537=VERTEX_POINT ( 'NONE', #8166 ) ;
#11555=DIRECTION ( 'NONE',  ( 0.000000000000000000, 0.000000000000000000, -1.000000000000000000 ) ) ;
#11559=LINE ( 'NONE', #6938, #2795 ) ;
#11606=CIRCLE ( 'NONE', #2835, 30.00000000000000711 ) ;
#11638=LINE ( 'NONE', #11513, #11687 ) ;
#11687=VECTOR ( 'NONE', #11451, 1000.000000000000000 ) ;
#11723=AXIS2_PLACEMENT_3D ( 'NONE', #2647, #8313, #2767 ) ;
#11731=EDGE_CURVE ( 'NONE', #3140, #5735, #367, .T. ) ;
#11749=PLANE ( 'NONE',  #1102 ) ;
#11826=EDGE_CURVE ( 'NONE', #1374, #6508, #12155, .T. ) ;
#11839=ORIENTED_EDGE ( 'NONE', *, *, #5598, .F. ) ;
#11875=FACE_OUTER_BOUND ( 'NONE', #2831, .T. ) ;
#11876=CARTESIAN_POINT ( 'NONE',  ( -25.00000000000000000, 570.2996408614167194, -88.00000000000000000 ) ) ;
#11882=DIRECTION ( 'NONE',  ( 0.000000000000000000, 1.000000000000000000, 0.000000000000000000 ) ) ;
#11910=DIRECTION ( 'NONE',  ( -0.000000000000000000, -1.000000000000000000, -0.000000000000000000 ) ) ;
#11915=EDGE_CURVE ( 'NONE', #3006, #6671, #8278, .T. ) ;
#11973=CARTESIAN_POINT ( 'NONE',  ( 25.00000000000000355, 570.2996408614167194, -90.00000000000000000 ) ) ;
#11996=DIRECTION ( 'NONE',  ( 1.000000000000000000, 0.000000000000000000, -0.000000000000000000 ) ) ;
#12004=DIRECTION ( 'NONE',  ( -0.000000000000000000, -1.000000000000000000, -0.000000000000000000 ) ) ;
#12064=AXIS2_PLACEMENT_3D ( 'NONE', #6649, #1848, #5601 ) ;
#12071=CLOSED_SHELL ( 'NONE', ( #9280, #2466, #6770, #6104, #3969, #1741 ) ) ;
#12155=CIRCLE ( 'NONE', #5782, 45.00000000000000000 ) ;
#12190=CARTESIAN_POINT ( 'NONE',  ( -25.00000000000000000, 570.2996408614167194, -90.00000000000000000 ) ) ;
#12278=APPLICATION_CONTEXT ( 'automotive_design' ) ;
#12287=CARTESIAN_POINT ( 'NONE',  ( 25.00000000000000000, 347.0000000000000568, -88.00000000000000000 ) ) ;
#12319=PLANE ( 'NONE',  #6424 ) ;
#12320=DIRECTION ( 'NONE',  ( 0.000000000000000000, 0.000000000000000000, 1.000000000000000000 ) ) ;
#12322=CIRCLE ( 'NONE', #11723, 28.00000000000000355 ) ;
ENDSEC;
END-ISO-10303-21;
